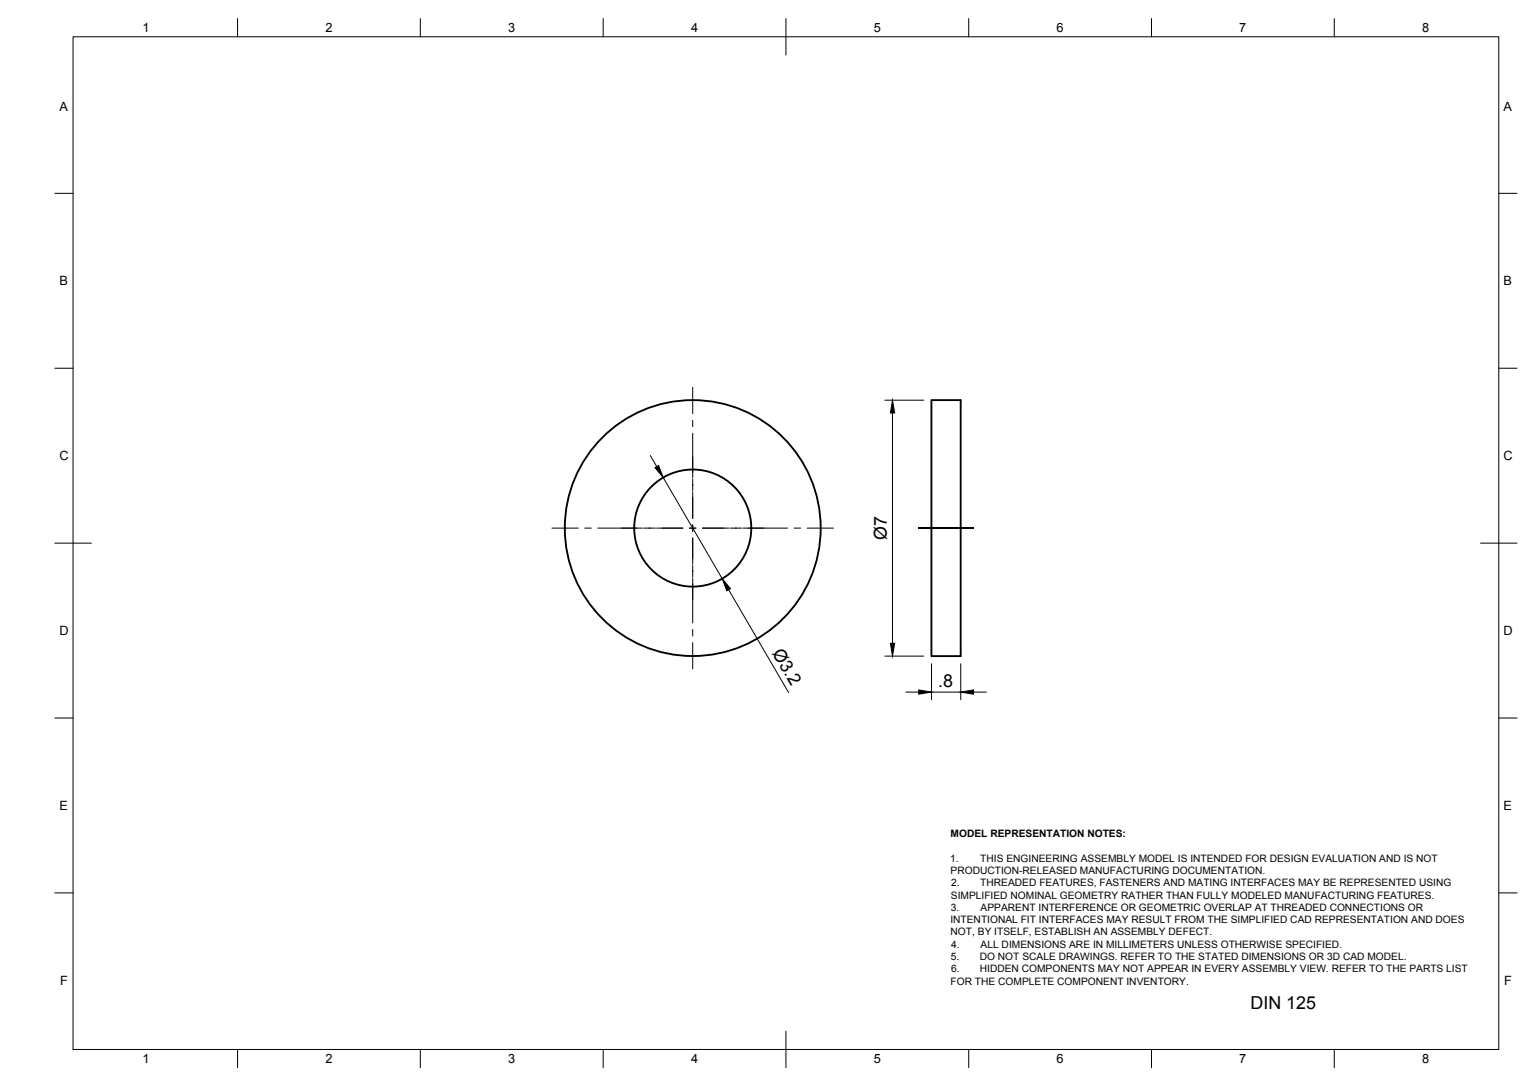
ISO-10303-21;
HEADER;
/* Generated by software containing ST-Developer
 * from STEP Tools, Inc. (www.steptools.com) 
 */

FILE_DESCRIPTION(
/* description */ ('STEP AP214'),
/* implementation_level */ '2;1');

FILE_NAME(
/* name */ 'DIN 125.step',
/* time_stamp */ '2026-10-07T12:18:07-07:00',
/* author */ (''),
/* organization */ (''),
/* preprocessor_version */ 'ST-DEVELOPER v20.2',
/* originating_system */ 'Autodesk Translation Framework v15.15.0.0',
/* authorisation */ '');

FILE_SCHEMA (('AUTOMOTIVE_DESIGN { 1 0 10303 214 3 1 1 }'));
ENDSEC;

DATA;
#10=MECHANICAL_DESIGN_GEOMETRIC_PRESENTATION_REPRESENTATION('',(#131),#62974);
#107=SHAPE_REPRESENTATION_RELATIONSHIP('SRR','None',#63030,#119);
#119=ADVANCED_BREP_SHAPE_REPRESENTATION('',(#143),#62971);
#131=STYLED_ITEM('',(#63090),#143);
#143=MANIFOLD_SOLID_BREP('Body1',#15201);
#275=FACE_BOUND('',#5465,.T.);
#276=FACE_BOUND('',#5467,.T.);
#714=PLANE('',#16863);
#715=PLANE('',#16864);
#2205=LINE('',#62646,#3398);
#2206=LINE('',#62652,#3399);
#3398=VECTOR('',#21148,3.5);
#3399=VECTOR('',#21155,1.6);
#3684=CYLINDRICAL_SURFACE('',#16857,3.5);
#3685=CYLINDRICAL_SURFACE('',#16860,1.6);
#4514=FACE_OUTER_BOUND('',#5462,.T.);
#4515=FACE_OUTER_BOUND('',#5463,.T.);
#4516=FACE_OUTER_BOUND('',#5464,.T.);
#4517=FACE_OUTER_BOUND('',#5466,.T.);
#5462=EDGE_LOOP('',(#14057,#14058,#14059,#14060));
#5463=EDGE_LOOP('',(#14061,#14062,#14063,#14064));
#5464=EDGE_LOOP('',(#14065));
#5465=EDGE_LOOP('',(#14066));
#5466=EDGE_LOOP('',(#14067));
#5467=EDGE_LOOP('',(#14068));
#6182=CIRCLE('',#16858,3.5);
#6183=CIRCLE('',#16859,3.5);
#6184=CIRCLE('',#16861,1.6);
#6185=CIRCLE('',#16862,1.6);
#7560=VERTEX_POINT('',#62643);
#7561=VERTEX_POINT('',#62645);
#7562=VERTEX_POINT('',#62649);
#7563=VERTEX_POINT('',#62651);
#9735=EDGE_CURVE('',#7560,#7560,#6182,.T.);
#9736=EDGE_CURVE('',#7560,#7561,#2205,.T.);
#9737=EDGE_CURVE('',#7561,#7561,#6183,.T.);
#9738=EDGE_CURVE('',#7562,#7562,#6184,.T.);
#9739=EDGE_CURVE('',#7562,#7563,#2206,.T.);
#9740=EDGE_CURVE('',#7563,#7563,#6185,.T.);
#14057=ORIENTED_EDGE('',*,*,#9735,.F.);
#14058=ORIENTED_EDGE('',*,*,#9736,.T.);
#14059=ORIENTED_EDGE('',*,*,#9737,.T.);
#14060=ORIENTED_EDGE('',*,*,#9736,.F.);
#14061=ORIENTED_EDGE('',*,*,#9738,.F.);
#14062=ORIENTED_EDGE('',*,*,#9739,.T.);
#14063=ORIENTED_EDGE('',*,*,#9740,.F.);
#14064=ORIENTED_EDGE('',*,*,#9739,.F.);
#14065=ORIENTED_EDGE('',*,*,#9737,.F.);
#14066=ORIENTED_EDGE('',*,*,#9738,.T.);
#14067=ORIENTED_EDGE('',*,*,#9735,.T.);
#14068=ORIENTED_EDGE('',*,*,#9740,.T.);
#15149=ADVANCED_FACE('',(#4514),#3684,.T.);
#15150=ADVANCED_FACE('',(#4515),#3685,.F.);
#15151=ADVANCED_FACE('',(#4516,#275),#714,.F.);
#15152=ADVANCED_FACE('',(#4517,#276),#715,.T.);
#15201=CLOSED_SHELL('',(#15149,#15150,#15151,#15152));
#16856=AXIS2_PLACEMENT_3D('',#62641,#21142,#21143);
#16857=AXIS2_PLACEMENT_3D('',#62642,#21144,#21145);
#16858=AXIS2_PLACEMENT_3D('',#62644,#21146,#21147);
#16859=AXIS2_PLACEMENT_3D('',#62647,#21149,#21150);
#16860=AXIS2_PLACEMENT_3D('',#62648,#21151,#21152);
#16861=AXIS2_PLACEMENT_3D('',#62650,#21153,#21154);
#16862=AXIS2_PLACEMENT_3D('',#62653,#21156,#21157);
#16863=AXIS2_PLACEMENT_3D('',#62654,#21158,#21159);
#16864=AXIS2_PLACEMENT_3D('',#62655,#21160,#21161);
#21142=DIRECTION('axis',(0.,0.,1.));
#21143=DIRECTION('refdir',(1.,0.,0.));
#21144=DIRECTION('center_axis',(1.,-1.E-15,0.));
#21145=DIRECTION('ref_axis',(9.91270557701032E-31,9.91270557701032E-16,
1.));
#21146=DIRECTION('center_axis',(1.,-1.E-15,0.));
#21147=DIRECTION('ref_axis',(9.91270557701032E-31,9.91270557701032E-16,
1.));
#21148=DIRECTION('',(-1.,1.E-15,0.));
#21149=DIRECTION('center_axis',(1.,-1.E-15,0.));
#21150=DIRECTION('ref_axis',(9.91270557701032E-31,9.91270557701032E-16,
1.));
#21151=DIRECTION('center_axis',(1.,-1.E-15,0.));
#21152=DIRECTION('ref_axis',(0.,0.,1.));
#21153=DIRECTION('center_axis',(1.,-1.E-15,0.));
#21154=DIRECTION('ref_axis',(0.,0.,1.));
#21155=DIRECTION('',(1.,-1.E-15,0.));
#21156=DIRECTION('center_axis',(-1.,1.E-15,0.));
#21157=DIRECTION('ref_axis',(0.,0.,-1.));
#21158=DIRECTION('center_axis',(1.,-1.E-15,0.));
#21159=DIRECTION('ref_axis',(-1.E-15,-1.,1.E-15));
#21160=DIRECTION('center_axis',(1.,-1.E-15,0.));
#21161=DIRECTION('ref_axis',(-1.E-15,-1.,1.E-15));
#62641=CARTESIAN_POINT('',(0.,0.,0.));
#62642=CARTESIAN_POINT('Origin',(35.8,21.,6.000000094481));
#62643=CARTESIAN_POINT('',(35.8,21.,2.500000094481));
#62644=CARTESIAN_POINT('Origin',(35.8,21.,6.000000094481));
#62645=CARTESIAN_POINT('',(35.,21.,2.500000094481));
#62646=CARTESIAN_POINT('',(35.8,21.,2.500000094481));
#62647=CARTESIAN_POINT('Origin',(35.,21.,6.000000094481));
#62648=CARTESIAN_POINT('Origin',(36.41,21.,6.000000094481));
#62649=CARTESIAN_POINT('',(35.,21.,4.400000094481));
#62650=CARTESIAN_POINT('Origin',(35.,21.,6.000000094481));
#62651=CARTESIAN_POINT('',(35.8,21.,4.400000094481));
#62652=CARTESIAN_POINT('',(36.41,21.,4.400000094481));
#62653=CARTESIAN_POINT('Origin',(35.8,21.,6.000000094481));
#62654=CARTESIAN_POINT('Origin',(35.,21.,6.000000094481));
#62655=CARTESIAN_POINT('Origin',(35.8,21.,6.000000094481));
#62957=UNCERTAINTY_MEASURE_WITH_UNIT(LENGTH_MEASURE(0.01),#62975,
'DISTANCE_ACCURACY_VALUE',
'Maximum model space distance between geometric entities at asserted c
onnectivities');
#62960=UNCERTAINTY_MEASURE_WITH_UNIT(LENGTH_MEASURE(0.01),#62975,
'DISTANCE_ACCURACY_VALUE',
'Maximum model space distance between geometric entities at asserted c
onnectivities');
#62971=(
GEOMETRIC_REPRESENTATION_CONTEXT(3)
GLOBAL_UNCERTAINTY_ASSIGNED_CONTEXT((#62957))
GLOBAL_UNIT_ASSIGNED_CONTEXT((#62975,#62977,#62978))
REPRESENTATION_CONTEXT('','3D')
);
#62974=(
GEOMETRIC_REPRESENTATION_CONTEXT(3)
GLOBAL_UNCERTAINTY_ASSIGNED_CONTEXT((#62960))
GLOBAL_UNIT_ASSIGNED_CONTEXT((#62975,#62977,#62978))
REPRESENTATION_CONTEXT('','3D')
);
#62975=(
LENGTH_UNIT()
NAMED_UNIT(*)
SI_UNIT(.MILLI.,.METRE.)
);
#62977=(
NAMED_UNIT(*)
PLANE_ANGLE_UNIT()
SI_UNIT($,.RADIAN.)
);
#62978=(
NAMED_UNIT(*)
SI_UNIT($,.STERADIAN.)
SOLID_ANGLE_UNIT()
);
#62989=SHAPE_DEFINITION_REPRESENTATION(#63002,#63030);
#63002=PRODUCT_DEFINITION_SHAPE('',$,#63044);
#63030=SHAPE_REPRESENTATION('',(#16856),#62971);
#63033=PRODUCT_DEFINITION_CONTEXT('part definition',#63074,'design');
#63044=PRODUCT_DEFINITION('DIN 125','DIN 125',#63057,#63033);
#63057=PRODUCT_DEFINITION_FORMATION('',$,#63086);
#63074=APPLICATION_CONTEXT(
'Core Data for Automotive Mechanical Design Process');
#63075=PRODUCT_CONTEXT('part definition',#63074,'mechanical');
#63086=PRODUCT('DIN 125','DIN 125',$,(#63075));
#63090=PRESENTATION_STYLE_ASSIGNMENT((#63092));
#63092=SURFACE_STYLE_USAGE(.BOTH.,#63094);
#63094=SURFACE_SIDE_STYLE('',(#63096));
#63096=SURFACE_STYLE_FILL_AREA(#63098);
#63098=FILL_AREA_STYLE('Opaque(202,209,238)',(#63100));
#63100=FILL_AREA_STYLE_COLOUR('Opaque(202,209,238)',#63102);
#63102=COLOUR_RGB('Opaque(202,209,238)', 0.66274510, 0.83137255, 0.94901961);
ENDSEC;
END-ISO-10303-21;
